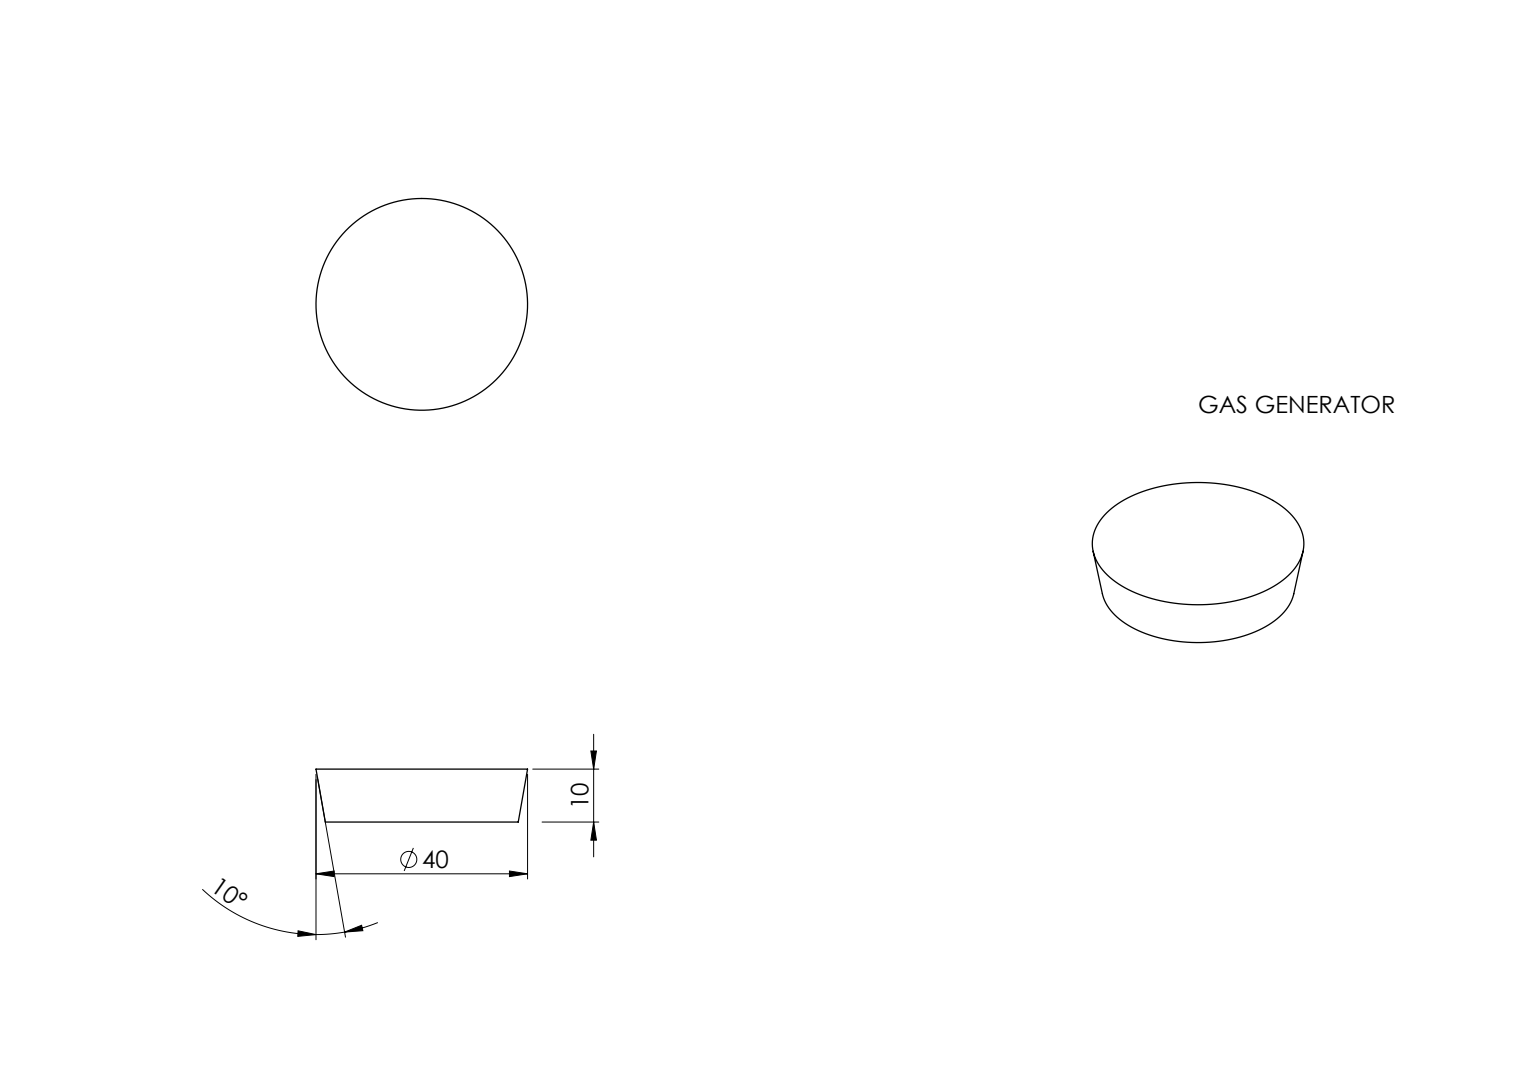
ISO-10303-21;
HEADER;
FILE_DESCRIPTION (('STEP AP214'),
    '1' );
FILE_NAME ('gas generator.step',
    '2026-10-24T15:06:47',
    ( '' ),
    ( '' ),
    'SwSTEP 2.0',
    'SolidWorks 2026',
    '' );
FILE_SCHEMA (( 'AUTOMOTIVE_DESIGN' ));
ENDSEC;

DATA;
#33=AXIS2_PLACEMENT_3D ( 'NONE', #2920, #5329, #6943 ) ;
#49=UNCERTAINTY_MEASURE_WITH_UNIT (LENGTH_MEASURE( 1.000000000000000082E-05 ), #5358, 'distance_accuracy_value', 'NONE');
#53=CARTESIAN_POINT ( 'NONE',  ( 0.000000000000000000, 85.00000000000000000, -20.00000000000000000 ) ) ;
#59=ORIENTED_EDGE ( 'NONE', *, *, #4217, .F. ) ;
#80=EDGE_CURVE ( 'NONE', #2765, #6040, #6971, .T. ) ;
#126=ORIENTED_EDGE ( 'NONE', *, *, #1417, .F. ) ;
#275=CARTESIAN_POINT ( 'NONE',  ( 0.000000000000000000, 75.00000000000001421, 0.000000000000000000 ) ) ;
#431=CONICAL_SURFACE ( 'NONE', #6456, 20.00000000000000000, 0.1745329251994333364 ) ;
#539=SURFACE_STYLE_FILL_AREA ( #8546 ) ;
#614=VECTOR ( 'NONE', #3685, 1000.000000000000000 ) ;
#686=DIRECTION ( 'NONE',  ( -2.126576849575776229E-17, 0.9848077530122080203, 0.1736481776669307198 ) ) ;
#725=( NAMED_UNIT ( * ) PLANE_ANGLE_UNIT ( ) SI_UNIT ( $, .RADIAN. ) );
#798=( GEOMETRIC_REPRESENTATION_CONTEXT ( 3 ) GLOBAL_UNCERTAINTY_ASSIGNED_CONTEXT ( ( #8646 ) ) GLOBAL_UNIT_ASSIGNED_CONTEXT ( ( #7893, #725, #8735 ) ) REPRESENTATION_CONTEXT ( 'NONE', 'WORKASPACE' ) );
#846=PRODUCT_DEFINITION_SHAPE ( 'NONE', 'NONE',  #4215 ) ;
#862=ORIENTED_EDGE ( 'NONE', *, *, #2814, .T. ) ;
#903=STYLED_ITEM ( 'NONE', ( #2100 ), #7366 ) ;
#952=DIRECTION ( 'NONE',  ( 0.000000000000000000, 0.000000000000000000, -1.000000000000000000 ) ) ;
#995=ADVANCED_FACE ( 'NONE', ( #8137 ), #431, .T. ) ;
#1045=AXIS2_PLACEMENT_3D ( 'NONE', #9396, #9454, #10292 ) ;
#1085=DIRECTION ( 'NONE',  ( 0.000000000000000000, 0.000000000000000000, -1.000000000000000000 ) ) ;
#1087=ADVANCED_FACE ( 'NONE', ( #2045 ), #3629, .T. ) ;
#1162=DIRECTION ( 'NONE',  ( 0.000000000000000000, -1.000000000000000000, 0.000000000000000000 ) ) ;
#1248=PRODUCT_CONTEXT ( 'NONE', #5122, 'mechanical' ) ;
#1370=( NAMED_UNIT ( * ) PLANE_ANGLE_UNIT ( ) SI_UNIT ( $, .RADIAN. ) );
#1417=EDGE_CURVE ( 'NONE', #6040, #2765, #7542, .T. ) ;
#1457=PLANE ( 'NONE',  #33 ) ;
#1584=SHAPE_REPRESENTATION ( 'gas generator', ( #5055 ), #5746 ) ;
#1613=EDGE_LOOP ( 'NONE', ( #4097, #59 ) ) ;
#1673=ADVANCED_FACE ( 'NONE', ( #5207 ), #1457, .F. ) ;
#1964=CARTESIAN_POINT ( 'NONE',  ( 0.000000000000000000, 85.00000000000000000, 0.000000000000000000 ) ) ;
#2045=FACE_OUTER_BOUND ( 'NONE', #5499, .T. ) ;
#2100=PRESENTATION_STYLE_ASSIGNMENT (( #9266 ) ) ;
#2337=ORIENTED_EDGE ( 'NONE', *, *, #3309, .T. ) ;
#2397=VECTOR ( 'NONE', #686, 1000.000000000000000 ) ;
#2461=PRODUCT_DEFINITION_CONTEXT ( 'detailed design', #2595, 'design' ) ;
#2595=APPLICATION_CONTEXT ( 'automotive_design' ) ;
#2723=CARTESIAN_POINT ( 'NONE',  ( 0.000000000000000000, 75.00000000000001421, -18.23673019291534558 ) ) ;
#2765=VERTEX_POINT ( 'NONE', #2723 ) ;
#2814=EDGE_CURVE ( 'NONE', #6040, #7000, #6643, .T. ) ;
#2920=CARTESIAN_POINT ( 'NONE',  ( 0.000000000000000000, 85.00000000000000000, 0.000000000000000000 ) ) ;
#3016=VERTEX_POINT ( 'NONE', #53 ) ;
#3039=ORIENTED_EDGE ( 'NONE', *, *, #80, .F. ) ;
#3059=AXIS2_PLACEMENT_3D ( 'NONE', #5619, #8121, #952 ) ;
#3309=EDGE_CURVE ( 'NONE', #3016, #7000, #9395, .T. ) ;
#3392=EDGE_LOOP ( 'NONE', ( #8665, #3039, #9271, #2337 ) ) ;
#3629=PLANE ( 'NONE',  #9470 ) ;
#3685=DIRECTION ( 'NONE',  ( 0.000000000000000000, 0.9848077530122080203, -0.1736481776669307198 ) ) ;
#4060=CARTESIAN_POINT ( 'NONE',  ( 0.000000000000000000, 85.00000000000000000, 0.000000000000000000 ) ) ;
#4089=ORIENTED_EDGE ( 'NONE', *, *, #4217, .T. ) ;
#4097=ORIENTED_EDGE ( 'NONE', *, *, #3309, .F. ) ;
#4154=DIRECTION ( 'NONE',  ( 0.000000000000000000, 0.000000000000000000, 1.000000000000000000 ) ) ;
#4159=DIRECTION ( 'NONE',  ( -0.000000000000000000, 1.000000000000000000, -0.000000000000000000 ) ) ;
#4215=PRODUCT_DEFINITION ( 'UNKNOWN', '', #6632, #2461 ) ;
#4217=EDGE_CURVE ( 'NONE', #7000, #3016, #4249, .T. ) ;
#4249=CIRCLE ( 'NONE', #5247, 20.00000000000000000 ) ;
#4344=CARTESIAN_POINT ( 'NONE',  ( 0.000000000000000000, 75.00000000000001421, 0.000000000000000000 ) ) ;
#4620=( NAMED_UNIT ( * ) SI_UNIT ( $, .STERADIAN. ) SOLID_ANGLE_UNIT ( ) );
#5055=AXIS2_PLACEMENT_3D ( 'NONE', #9842, #4154, #9744 ) ;
#5056=FACE_OUTER_BOUND ( 'NONE', #6539, .T. ) ;
#5122=APPLICATION_CONTEXT ( 'automotive_design' ) ;
#5207=FACE_OUTER_BOUND ( 'NONE', #1613, .T. ) ;
#5247=AXIS2_PLACEMENT_3D ( 'NONE', #9442, #7761, #6972 ) ;
#5329=DIRECTION ( 'NONE',  ( 0.000000000000000000, -1.000000000000000000, 0.000000000000000000 ) ) ;
#5358=( LENGTH_UNIT ( ) NAMED_UNIT ( * ) SI_UNIT ( .MILLI., .METRE. ) );
#5422=COLOUR_RGB ( '',0.8941176470588234615, 0.8941176470588234615, 0.8941176470588234615 ) ;
#5499=EDGE_LOOP ( 'NONE', ( #5673, #8460 ) ) ;
#5619=CARTESIAN_POINT ( 'NONE',  ( 0.000000000000000000, 75.00000000000001421, 0.000000000000000000 ) ) ;
#5673=ORIENTED_EDGE ( 'NONE', *, *, #80, .T. ) ;
#5708=CARTESIAN_POINT ( 'NONE',  ( -2.341324462030736955E-15, 75.00000000000001421, 18.23673019291534558 ) ) ;
#5746=( GEOMETRIC_REPRESENTATION_CONTEXT ( 3 ) GLOBAL_UNCERTAINTY_ASSIGNED_CONTEXT ( ( #49 ) ) GLOBAL_UNIT_ASSIGNED_CONTEXT ( ( #5358, #7644, #6805 ) ) REPRESENTATION_CONTEXT ( 'NONE', 'WORKASPACE' ) );
#5793=MECHANICAL_DESIGN_GEOMETRIC_PRESENTATION_REPRESENTATION('',(#7982),#798);
#6040=VERTEX_POINT ( 'NONE', #5708 ) ;
#6298=MANIFOLD_SOLID_BREP ( 'Boss-Extrude1', #8814 ) ;
#6318=AXIS2_PLACEMENT_3D ( 'NONE', #4344, #6748, #9109 ) ;
#6415=DIRECTION ( 'NONE',  ( 0.000000000000000000, 0.000000000000000000, -1.000000000000000000 ) ) ;
#6456=AXIS2_PLACEMENT_3D ( 'NONE', #4060, #4159, #6415 ) ;
#6539=EDGE_LOOP ( 'NONE', ( #126, #862, #4089, #6681 ) ) ;
#6632=PRODUCT_DEFINITION_FORMATION_WITH_SPECIFIED_SOURCE ( 'ANY', '', #7772, .NOT_KNOWN. ) ;
#6643=LINE ( 'NONE', #6962, #2397 ) ;
#6681=ORIENTED_EDGE ( 'NONE', *, *, #8781, .F. ) ;
#6748=DIRECTION ( 'NONE',  ( 0.000000000000000000, -1.000000000000000000, 0.000000000000000000 ) ) ;
#6805=( NAMED_UNIT ( * ) SI_UNIT ( $, .STERADIAN. ) SOLID_ANGLE_UNIT ( ) );
#6858=FILL_AREA_STYLE_COLOUR ( '', #5422 ) ;
#6943=DIRECTION ( 'NONE',  ( 0.000000000000000000, -0.000000000000000000, -1.000000000000000000 ) ) ;
#6962=CARTESIAN_POINT ( 'NONE',  ( -2.449293598294706513E-15, 85.00000000000000000, 20.00000000000000000 ) ) ;
#6971=CIRCLE ( 'NONE', #6318, 18.23673019291534558 ) ;
#6972=DIRECTION ( 'NONE',  ( 0.000000000000000000, 0.000000000000000000, -1.000000000000000000 ) ) ;
#7000=VERTEX_POINT ( 'NONE', #10217 ) ;
#7171=ADVANCED_FACE ( 'NONE', ( #5056 ), #9507, .T. ) ;
#7366=ADVANCED_BREP_SHAPE_REPRESENTATION ( '', ( #6298, #5055 ), #5746 ) ;
#7519=SHAPE_DEFINITION_REPRESENTATION ( #846, #1584 ) ;
#7542=CIRCLE ( 'NONE', #3059, 18.23673019291534558 ) ;
#7644=( NAMED_UNIT ( * ) PLANE_ANGLE_UNIT ( ) SI_UNIT ( $, .RADIAN. ) );
#7702=SHAPE_REPRESENTATION_RELATIONSHIP ( 'NONE' , 'NONE' ,  #1584, #7366 ) ;
#7761=DIRECTION ( 'NONE',  ( 0.000000000000000000, -1.000000000000000000, 0.000000000000000000 ) ) ;
#7772=PRODUCT ( 'gas generator', 'gas generator', '', ( #1248 ) ) ;
#7893=( LENGTH_UNIT ( ) NAMED_UNIT ( * ) SI_UNIT ( .MILLI., .METRE. ) );
#7982=STYLED_ITEM('',(#10394),#6298);
#8121=DIRECTION ( 'NONE',  ( 0.000000000000000000, -1.000000000000000000, 0.000000000000000000 ) ) ;
#8137=FACE_OUTER_BOUND ( 'NONE', #3392, .T. ) ;
#8357=DIRECTION ( 'NONE',  ( -0.000000000000000000, 1.000000000000000000, -0.000000000000000000 ) ) ;
#8460=ORIENTED_EDGE ( 'NONE', *, *, #1417, .T. ) ;
#8490=( LENGTH_UNIT ( ) NAMED_UNIT ( * ) SI_UNIT ( .MILLI., .METRE. ) );
#8501=LINE ( 'NONE', #10011, #614 ) ;
#8546=FILL_AREA_STYLE ('',( #6858 ) ) ;
#8646=UNCERTAINTY_MEASURE_WITH_UNIT (LENGTH_MEASURE( 1.000000000000000082E-05 ), #7893, 'distance_accuracy_value', 'NONE');
#8665=ORIENTED_EDGE ( 'NONE', *, *, #2814, .F. ) ;
#8735=( NAMED_UNIT ( * ) SI_UNIT ( $, .STERADIAN. ) SOLID_ANGLE_UNIT ( ) );
#8781=EDGE_CURVE ( 'NONE', #2765, #3016, #8501, .T. ) ;
#8814=CLOSED_SHELL ( 'NONE', ( #7171, #995, #1087, #1673 ) ) ;
#8847=UNCERTAINTY_MEASURE_WITH_UNIT (LENGTH_MEASURE( 1.000000000000000082E-05 ), #8490, 'distance_accuracy_value', 'NONE');
#8921=( GEOMETRIC_REPRESENTATION_CONTEXT ( 3 ) GLOBAL_UNCERTAINTY_ASSIGNED_CONTEXT ( ( #8847 ) ) GLOBAL_UNIT_ASSIGNED_CONTEXT ( ( #8490, #1370, #4620 ) ) REPRESENTATION_CONTEXT ( 'NONE', 'WORKASPACE' ) );
#8985=AXIS2_PLACEMENT_3D ( 'NONE', #1964, #8357, #1085 ) ;
#9109=DIRECTION ( 'NONE',  ( 0.000000000000000000, 0.000000000000000000, -1.000000000000000000 ) ) ;
#9266=SURFACE_STYLE_USAGE ( .BOTH. , #10054 ) ;
#9271=ORIENTED_EDGE ( 'NONE', *, *, #8781, .T. ) ;
#9395=CIRCLE ( 'NONE', #1045, 20.00000000000000000 ) ;
#9396=CARTESIAN_POINT ( 'NONE',  ( 0.000000000000000000, 85.00000000000000000, 0.000000000000000000 ) ) ;
#9442=CARTESIAN_POINT ( 'NONE',  ( 0.000000000000000000, 85.00000000000000000, 0.000000000000000000 ) ) ;
#9454=DIRECTION ( 'NONE',  ( 0.000000000000000000, -1.000000000000000000, 0.000000000000000000 ) ) ;
#9470=AXIS2_PLACEMENT_3D ( 'NONE', #275, #1162, #9954 ) ;
#9507=CONICAL_SURFACE ( 'NONE', #8985, 20.00000000000000000, 0.1745329251994333364 ) ;
#9744=DIRECTION ( 'NONE',  ( 1.000000000000000000, 0.000000000000000000, 0.000000000000000000 ) ) ;
#9749=MECHANICAL_DESIGN_GEOMETRIC_PRESENTATION_REPRESENTATION('',(#903),#8921);
#9842=CARTESIAN_POINT ( 'NONE',  ( 0.000000000000000000, 0.000000000000000000, 0.000000000000000000 ) ) ;
#9954=DIRECTION ( 'NONE',  ( 0.000000000000000000, -0.000000000000000000, -1.000000000000000000 ) ) ;
#10011=CARTESIAN_POINT ( 'NONE',  ( 0.000000000000000000, 85.00000000000000000, -20.00000000000000000 ) ) ;
#10054=SURFACE_SIDE_STYLE ('',( #539 ) ) ;
#10217=CARTESIAN_POINT ( 'NONE',  ( -2.449293598294706513E-15, 85.00000000000000000, 20.00000000000000000 ) ) ;
#10292=DIRECTION ( 'NONE',  ( 0.000000000000000000, 0.000000000000000000, -1.000000000000000000 ) ) ;
#10388=COLOUR_RGB('Sky Blue',0.24,0.69,0.87);
#10389=FILL_AREA_STYLE_COLOUR('',#10388);
#10390=FILL_AREA_STYLE('',(#10389));
#10391=SURFACE_STYLE_FILL_AREA(#10390);
#10392=SURFACE_SIDE_STYLE('',(#10391));
#10393=SURFACE_STYLE_USAGE(.BOTH.,#10392);
#10394=PRESENTATION_STYLE_ASSIGNMENT((#10393));
ENDSEC;
END-ISO-10303-21;
